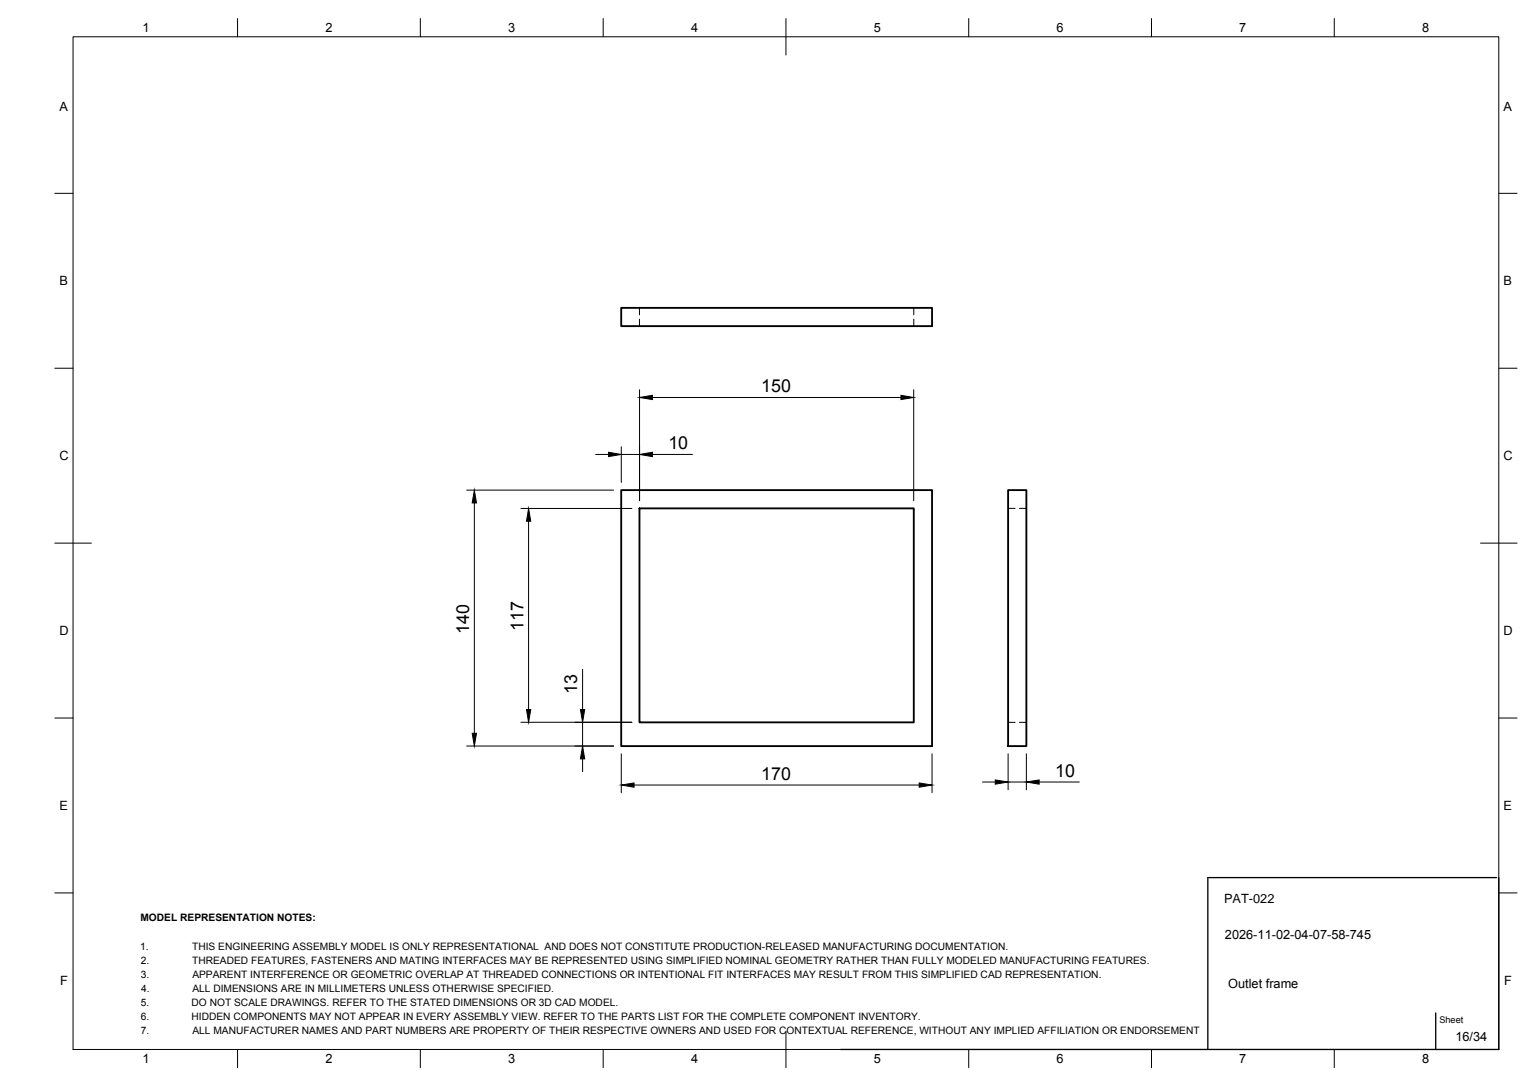
ISO-10303-21;
HEADER;
/* Generated by software containing ST-Developer
 * from STEP Tools, Inc. (www.steptools.com) 
 */

FILE_DESCRIPTION(
/* description */ ('Chute with adjustable gate'),
/* implementation_level */ '2;1');

FILE_NAME(
/* name */ 'Outlet frame.step',
/* time_stamp */ '2026-10-27T10:52:28-07:00',
/* author */ (''),
/* organization */ (''),
/* preprocessor_version */ 'ST-DEVELOPER v20.2',
/* originating_system */ 'Autodesk Translation Framework v15.17.0.0',
/* authorisation */ '');

FILE_SCHEMA (('AUTOMOTIVE_DESIGN { 1 0 10303 214 3 1 1 }'));
ENDSEC;

DATA;
#10=MECHANICAL_DESIGN_GEOMETRIC_PRESENTATION_REPRESENTATION('',(#425),#13094);
#361=SHAPE_REPRESENTATION_RELATIONSHIP('SRR','None',#13262,#393);
#393=ADVANCED_BREP_SHAPE_REPRESENTATION('',(#457),#13071);
#425=STYLED_ITEM('',(#13474),#457);
#457=MANIFOLD_SOLID_BREP('Body1',#7608);
#516=FACE_BOUND('',#1482,.T.);
#517=FACE_BOUND('',#1484,.T.);
#668=PLANE('',#8150);
#669=PLANE('',#8151);
#670=PLANE('',#8152);
#671=PLANE('',#8153);
#672=PLANE('',#8154);
#673=PLANE('',#8155);
#674=PLANE('',#8156);
#675=PLANE('',#8157);
#676=PLANE('',#8158);
#677=PLANE('',#8159);
#1016=FACE_OUTER_BOUND('',#1473,.T.);
#1017=FACE_OUTER_BOUND('',#1474,.T.);
#1018=FACE_OUTER_BOUND('',#1475,.T.);
#1019=FACE_OUTER_BOUND('',#1476,.T.);
#1020=FACE_OUTER_BOUND('',#1477,.T.);
#1021=FACE_OUTER_BOUND('',#1478,.T.);
#1022=FACE_OUTER_BOUND('',#1479,.T.);
#1023=FACE_OUTER_BOUND('',#1480,.T.);
#1024=FACE_OUTER_BOUND('',#1481,.T.);
#1025=FACE_OUTER_BOUND('',#1483,.T.);
#1473=EDGE_LOOP('',(#5618,#5619,#5620,#5621));
#1474=EDGE_LOOP('',(#5622,#5623,#5624,#5625));
#1475=EDGE_LOOP('',(#5626,#5627,#5628,#5629));
#1476=EDGE_LOOP('',(#5630,#5631,#5632,#5633));
#1477=EDGE_LOOP('',(#5634,#5635,#5636,#5637));
#1478=EDGE_LOOP('',(#5638,#5639,#5640,#5641));
#1479=EDGE_LOOP('',(#5642,#5643,#5644,#5645));
#1480=EDGE_LOOP('',(#5646,#5647,#5648,#5649));
#1481=EDGE_LOOP('',(#5650,#5651,#5652,#5653));
#1482=EDGE_LOOP('',(#5654,#5655,#5656,#5657));
#1483=EDGE_LOOP('',(#5658,#5659,#5660,#5661));
#1484=EDGE_LOOP('',(#5662,#5663,#5664,#5665));
#2028=LINE('',#11378,#2805);
#2029=LINE('',#11380,#2806);
#2030=LINE('',#11382,#2807);
#2031=LINE('',#11383,#2808);
#2032=LINE('',#11386,#2809);
#2033=LINE('',#11388,#2810);
#2034=LINE('',#11389,#2811);
#2035=LINE('',#11392,#2812);
#2036=LINE('',#11394,#2813);
#2037=LINE('',#11395,#2814);
#2038=LINE('',#11397,#2815);
#2039=LINE('',#11398,#2816);
#2040=LINE('',#11402,#2817);
#2041=LINE('',#11404,#2818);
#2042=LINE('',#11406,#2819);
#2043=LINE('',#11407,#2820);
#2044=LINE('',#11410,#2821);
#2045=LINE('',#11412,#2822);
#2046=LINE('',#11413,#2823);
#2047=LINE('',#11416,#2824);
#2048=LINE('',#11418,#2825);
#2049=LINE('',#11419,#2826);
#2050=LINE('',#11421,#2827);
#2051=LINE('',#11422,#2828);
#2805=VECTOR('',#9196,1.);
#2806=VECTOR('',#9197,1.);
#2807=VECTOR('',#9198,1.);
#2808=VECTOR('',#9199,1.);
#2809=VECTOR('',#9202,1.);
#2810=VECTOR('',#9203,1.);
#2811=VECTOR('',#9204,1.);
#2812=VECTOR('',#9207,1.);
#2813=VECTOR('',#9208,1.);
#2814=VECTOR('',#9209,1.);
#2815=VECTOR('',#9212,1.);
#2816=VECTOR('',#9213,1.);
#2817=VECTOR('',#9216,1.);
#2818=VECTOR('',#9217,1.);
#2819=VECTOR('',#9218,1.);
#2820=VECTOR('',#9219,1.);
#2821=VECTOR('',#9222,1.);
#2822=VECTOR('',#9223,1.);
#2823=VECTOR('',#9224,1.);
#2824=VECTOR('',#9227,1.);
#2825=VECTOR('',#9228,1.);
#2826=VECTOR('',#9229,1.);
#2827=VECTOR('',#9232,1.);
#2828=VECTOR('',#9233,1.);
#3737=VERTEX_POINT('',#11376);
#3738=VERTEX_POINT('',#11377);
#3739=VERTEX_POINT('',#11379);
#3740=VERTEX_POINT('',#11381);
#3741=VERTEX_POINT('',#11385);
#3742=VERTEX_POINT('',#11387);
#3743=VERTEX_POINT('',#11391);
#3744=VERTEX_POINT('',#11393);
#3745=VERTEX_POINT('',#11400);
#3746=VERTEX_POINT('',#11401);
#3747=VERTEX_POINT('',#11403);
#3748=VERTEX_POINT('',#11405);
#3749=VERTEX_POINT('',#11409);
#3750=VERTEX_POINT('',#11411);
#3751=VERTEX_POINT('',#11415);
#3752=VERTEX_POINT('',#11417);
#4442=EDGE_CURVE('',#3737,#3738,#2028,.T.);
#4443=EDGE_CURVE('',#3739,#3737,#2029,.T.);
#4444=EDGE_CURVE('',#3740,#3739,#2030,.T.);
#4445=EDGE_CURVE('',#3740,#3738,#2031,.T.);
#4446=EDGE_CURVE('',#3738,#3741,#2032,.T.);
#4447=EDGE_CURVE('',#3742,#3740,#2033,.T.);
#4448=EDGE_CURVE('',#3742,#3741,#2034,.T.);
#4449=EDGE_CURVE('',#3741,#3743,#2035,.T.);
#4450=EDGE_CURVE('',#3744,#3742,#2036,.T.);
#4451=EDGE_CURVE('',#3744,#3743,#2037,.T.);
#4452=EDGE_CURVE('',#3743,#3737,#2038,.T.);
#4453=EDGE_CURVE('',#3739,#3744,#2039,.T.);
#4454=EDGE_CURVE('',#3745,#3746,#2040,.T.);
#4455=EDGE_CURVE('',#3746,#3747,#2041,.T.);
#4456=EDGE_CURVE('',#3748,#3747,#2042,.T.);
#4457=EDGE_CURVE('',#3745,#3748,#2043,.T.);
#4458=EDGE_CURVE('',#3749,#3745,#2044,.T.);
#4459=EDGE_CURVE('',#3750,#3748,#2045,.T.);
#4460=EDGE_CURVE('',#3749,#3750,#2046,.T.);
#4461=EDGE_CURVE('',#3751,#3749,#2047,.T.);
#4462=EDGE_CURVE('',#3752,#3750,#2048,.T.);
#4463=EDGE_CURVE('',#3751,#3752,#2049,.T.);
#4464=EDGE_CURVE('',#3746,#3751,#2050,.T.);
#4465=EDGE_CURVE('',#3747,#3752,#2051,.T.);
#5618=ORIENTED_EDGE('',*,*,#4442,.F.);
#5619=ORIENTED_EDGE('',*,*,#4443,.F.);
#5620=ORIENTED_EDGE('',*,*,#4444,.F.);
#5621=ORIENTED_EDGE('',*,*,#4445,.T.);
#5622=ORIENTED_EDGE('',*,*,#4446,.F.);
#5623=ORIENTED_EDGE('',*,*,#4445,.F.);
#5624=ORIENTED_EDGE('',*,*,#4447,.F.);
#5625=ORIENTED_EDGE('',*,*,#4448,.T.);
#5626=ORIENTED_EDGE('',*,*,#4449,.F.);
#5627=ORIENTED_EDGE('',*,*,#4448,.F.);
#5628=ORIENTED_EDGE('',*,*,#4450,.F.);
#5629=ORIENTED_EDGE('',*,*,#4451,.T.);
#5630=ORIENTED_EDGE('',*,*,#4452,.F.);
#5631=ORIENTED_EDGE('',*,*,#4451,.F.);
#5632=ORIENTED_EDGE('',*,*,#4453,.F.);
#5633=ORIENTED_EDGE('',*,*,#4443,.T.);
#5634=ORIENTED_EDGE('',*,*,#4454,.T.);
#5635=ORIENTED_EDGE('',*,*,#4455,.T.);
#5636=ORIENTED_EDGE('',*,*,#4456,.F.);
#5637=ORIENTED_EDGE('',*,*,#4457,.F.);
#5638=ORIENTED_EDGE('',*,*,#4458,.T.);
#5639=ORIENTED_EDGE('',*,*,#4457,.T.);
#5640=ORIENTED_EDGE('',*,*,#4459,.F.);
#5641=ORIENTED_EDGE('',*,*,#4460,.F.);
#5642=ORIENTED_EDGE('',*,*,#4461,.T.);
#5643=ORIENTED_EDGE('',*,*,#4460,.T.);
#5644=ORIENTED_EDGE('',*,*,#4462,.F.);
#5645=ORIENTED_EDGE('',*,*,#4463,.F.);
#5646=ORIENTED_EDGE('',*,*,#4464,.T.);
#5647=ORIENTED_EDGE('',*,*,#4463,.T.);
#5648=ORIENTED_EDGE('',*,*,#4465,.F.);
#5649=ORIENTED_EDGE('',*,*,#4455,.F.);
#5650=ORIENTED_EDGE('',*,*,#4465,.T.);
#5651=ORIENTED_EDGE('',*,*,#4462,.T.);
#5652=ORIENTED_EDGE('',*,*,#4459,.T.);
#5653=ORIENTED_EDGE('',*,*,#4456,.T.);
#5654=ORIENTED_EDGE('',*,*,#4449,.T.);
#5655=ORIENTED_EDGE('',*,*,#4452,.T.);
#5656=ORIENTED_EDGE('',*,*,#4442,.T.);
#5657=ORIENTED_EDGE('',*,*,#4446,.T.);
#5658=ORIENTED_EDGE('',*,*,#4464,.F.);
#5659=ORIENTED_EDGE('',*,*,#4454,.F.);
#5660=ORIENTED_EDGE('',*,*,#4458,.F.);
#5661=ORIENTED_EDGE('',*,*,#4461,.F.);
#5662=ORIENTED_EDGE('',*,*,#4450,.T.);
#5663=ORIENTED_EDGE('',*,*,#4447,.T.);
#5664=ORIENTED_EDGE('',*,*,#4444,.T.);
#5665=ORIENTED_EDGE('',*,*,#4453,.T.);
#7284=ADVANCED_FACE('',(#1016),#668,.F.);
#7285=ADVANCED_FACE('',(#1017),#669,.F.);
#7286=ADVANCED_FACE('',(#1018),#670,.F.);
#7287=ADVANCED_FACE('',(#1019),#671,.F.);
#7288=ADVANCED_FACE('',(#1020),#672,.T.);
#7289=ADVANCED_FACE('',(#1021),#673,.T.);
#7290=ADVANCED_FACE('',(#1022),#674,.T.);
#7291=ADVANCED_FACE('',(#1023),#675,.T.);
#7292=ADVANCED_FACE('',(#1024,#516),#676,.T.);
#7293=ADVANCED_FACE('',(#1025,#517),#677,.F.);
#7608=CLOSED_SHELL('',(#7284,#7285,#7286,#7287,#7288,#7289,#7290,#7291,
#7292,#7293));
#8149=AXIS2_PLACEMENT_3D('',#11374,#9192,#9193);
#8150=AXIS2_PLACEMENT_3D('',#11375,#9194,#9195);
#8151=AXIS2_PLACEMENT_3D('',#11384,#9200,#9201);
#8152=AXIS2_PLACEMENT_3D('',#11390,#9205,#9206);
#8153=AXIS2_PLACEMENT_3D('',#11396,#9210,#9211);
#8154=AXIS2_PLACEMENT_3D('',#11399,#9214,#9215);
#8155=AXIS2_PLACEMENT_3D('',#11408,#9220,#9221);
#8156=AXIS2_PLACEMENT_3D('',#11414,#9225,#9226);
#8157=AXIS2_PLACEMENT_3D('',#11420,#9230,#9231);
#8158=AXIS2_PLACEMENT_3D('',#11423,#9234,#9235);
#8159=AXIS2_PLACEMENT_3D('',#11424,#9236,#9237);
#9192=DIRECTION('axis',(0.,0.,1.));
#9193=DIRECTION('refdir',(1.,0.,0.));
#9194=DIRECTION('center_axis',(0.,0.,-1.));
#9195=DIRECTION('ref_axis',(0.,1.,0.));
#9196=DIRECTION('',(0.,-1.,0.));
#9197=DIRECTION('',(1.,0.,0.));
#9198=DIRECTION('',(0.,1.,0.));
#9199=DIRECTION('',(1.,0.,0.));
#9200=DIRECTION('center_axis',(0.,-1.,0.));
#9201=DIRECTION('ref_axis',(0.,0.,-1.));
#9202=DIRECTION('',(0.,0.,1.));
#9203=DIRECTION('',(0.,0.,-1.));
#9204=DIRECTION('',(1.,0.,0.));
#9205=DIRECTION('center_axis',(0.,0.,1.));
#9206=DIRECTION('ref_axis',(0.,-1.,0.));
#9207=DIRECTION('',(0.,1.,0.));
#9208=DIRECTION('',(0.,-1.,0.));
#9209=DIRECTION('',(1.,0.,0.));
#9210=DIRECTION('center_axis',(0.,1.,0.));
#9211=DIRECTION('ref_axis',(0.,0.,1.));
#9212=DIRECTION('',(0.,0.,-1.));
#9213=DIRECTION('',(0.,0.,1.));
#9214=DIRECTION('center_axis',(0.,0.,1.));
#9215=DIRECTION('ref_axis',(0.,-1.,0.));
#9216=DIRECTION('',(0.,-1.,0.));
#9217=DIRECTION('',(1.,0.,0.));
#9218=DIRECTION('',(0.,-1.,0.));
#9219=DIRECTION('',(1.,0.,0.));
#9220=DIRECTION('center_axis',(0.,1.,0.));
#9221=DIRECTION('ref_axis',(0.,0.,1.));
#9222=DIRECTION('',(0.,0.,1.));
#9223=DIRECTION('',(0.,0.,1.));
#9224=DIRECTION('',(1.,0.,0.));
#9225=DIRECTION('center_axis',(0.,0.,-1.));
#9226=DIRECTION('ref_axis',(0.,1.,0.));
#9227=DIRECTION('',(0.,1.,0.));
#9228=DIRECTION('',(0.,1.,0.));
#9229=DIRECTION('',(1.,0.,0.));
#9230=DIRECTION('center_axis',(0.,-1.,0.));
#9231=DIRECTION('ref_axis',(0.,0.,-1.));
#9232=DIRECTION('',(0.,0.,-1.));
#9233=DIRECTION('',(0.,0.,-1.));
#9234=DIRECTION('center_axis',(1.,0.,0.));
#9235=DIRECTION('ref_axis',(0.,0.,-1.));
#9236=DIRECTION('center_axis',(1.,0.,0.));
#9237=DIRECTION('ref_axis',(0.,0.,-1.));
#11374=CARTESIAN_POINT('',(0.,0.,0.));
#11375=CARTESIAN_POINT('Origin',(-1.1,-7.5,4.3));
#11376=CARTESIAN_POINT('',(0.,7.5,4.3));
#11377=CARTESIAN_POINT('',(0.,-7.5,4.3));
#11378=CARTESIAN_POINT('',(0.,-3.75,4.3));
#11379=CARTESIAN_POINT('',(-1.,7.5,4.3));
#11380=CARTESIAN_POINT('',(-1.1,7.5,4.3));
#11381=CARTESIAN_POINT('',(-1.,-7.5,4.3));
#11382=CARTESIAN_POINT('',(-1.,-3.75,4.3));
#11383=CARTESIAN_POINT('',(-1.1,-7.5,4.3));
#11384=CARTESIAN_POINT('Origin',(-1.1,-7.5,16.));
#11385=CARTESIAN_POINT('',(0.,-7.5,16.));
#11386=CARTESIAN_POINT('',(0.,-7.5,13.));
#11387=CARTESIAN_POINT('',(-1.,-7.5,16.));
#11388=CARTESIAN_POINT('',(-1.,-7.5,13.));
#11389=CARTESIAN_POINT('',(-1.1,-7.5,16.));
#11390=CARTESIAN_POINT('Origin',(-1.1,7.5,16.));
#11391=CARTESIAN_POINT('',(0.,7.5,16.));
#11392=CARTESIAN_POINT('',(0.,3.75,16.));
#11393=CARTESIAN_POINT('',(-1.,7.5,16.));
#11394=CARTESIAN_POINT('',(-1.,3.75,16.));
#11395=CARTESIAN_POINT('',(-1.1,7.5,16.));
#11396=CARTESIAN_POINT('Origin',(-1.1,7.5,4.3));
#11397=CARTESIAN_POINT('',(0.,7.5,7.15));
#11398=CARTESIAN_POINT('',(-1.,7.5,7.15));
#11399=CARTESIAN_POINT('Origin',(-1.,8.5,17.));
#11400=CARTESIAN_POINT('',(-1.,8.5,17.));
#11401=CARTESIAN_POINT('',(-1.,-8.5,17.));
#11402=CARTESIAN_POINT('',(-1.,8.5,17.));
#11403=CARTESIAN_POINT('',(0.,-8.5,17.));
#11404=CARTESIAN_POINT('',(-1.,-8.5,17.));
#11405=CARTESIAN_POINT('',(0.,8.5,17.));
#11406=CARTESIAN_POINT('',(0.,8.5,17.));
#11407=CARTESIAN_POINT('',(-1.,8.5,17.));
#11408=CARTESIAN_POINT('Origin',(-1.,8.5,3.));
#11409=CARTESIAN_POINT('',(-1.,8.5,3.));
#11410=CARTESIAN_POINT('',(-1.,8.5,3.));
#11411=CARTESIAN_POINT('',(0.,8.5,3.));
#11412=CARTESIAN_POINT('',(0.,8.5,3.));
#11413=CARTESIAN_POINT('',(-1.,8.5,3.));
#11414=CARTESIAN_POINT('Origin',(-1.,-8.5,3.));
#11415=CARTESIAN_POINT('',(-1.,-8.5,3.));
#11416=CARTESIAN_POINT('',(-1.,-8.5,3.));
#11417=CARTESIAN_POINT('',(0.,-8.5,3.));
#11418=CARTESIAN_POINT('',(0.,-8.5,3.));
#11419=CARTESIAN_POINT('',(-1.,-8.5,3.));
#11420=CARTESIAN_POINT('Origin',(-1.,-8.5,17.));
#11421=CARTESIAN_POINT('',(-1.,-8.5,17.));
#11422=CARTESIAN_POINT('',(0.,-8.5,17.));
#11423=CARTESIAN_POINT('Origin',(0.,0.,10.));
#11424=CARTESIAN_POINT('Origin',(-1.,0.,10.));
#13034=UNCERTAINTY_MEASURE_WITH_UNIT(LENGTH_MEASURE(0.001),#13095,
'DISTANCE_ACCURACY_VALUE',
'Maximum model space distance between geometric entities at asserted c
onnectivities');
#13057=UNCERTAINTY_MEASURE_WITH_UNIT(LENGTH_MEASURE(0.001),#13095,
'DISTANCE_ACCURACY_VALUE',
'Maximum model space distance between geometric entities at asserted c
onnectivities');
#13071=(
GEOMETRIC_REPRESENTATION_CONTEXT(3)
GLOBAL_UNCERTAINTY_ASSIGNED_CONTEXT((#13034))
GLOBAL_UNIT_ASSIGNED_CONTEXT((#13095,#13097,#13098))
REPRESENTATION_CONTEXT('','3D')
);
#13094=(
GEOMETRIC_REPRESENTATION_CONTEXT(3)
GLOBAL_UNCERTAINTY_ASSIGNED_CONTEXT((#13057))
GLOBAL_UNIT_ASSIGNED_CONTEXT((#13095,#13097,#13098))
REPRESENTATION_CONTEXT('','3D')
);
#13095=(
LENGTH_UNIT()
NAMED_UNIT(*)
SI_UNIT(.CENTI.,.METRE.)
);
#13097=(
NAMED_UNIT(*)
PLANE_ANGLE_UNIT()
SI_UNIT($,.RADIAN.)
);
#13098=(
NAMED_UNIT(*)
SI_UNIT($,.STERADIAN.)
SOLID_ANGLE_UNIT()
);
#13112=SHAPE_DEFINITION_REPRESENTATION(#13148,#13262);
#13148=PRODUCT_DEFINITION_SHAPE('',$,#13299);
#13262=SHAPE_REPRESENTATION('',(#8149),#13071);
#13285=PRODUCT_DEFINITION_CONTEXT('part definition',#13395,'design');
#13299=PRODUCT_DEFINITION('Outlet frame','Outlet frame',#13335,#13285);
#13335=PRODUCT_DEFINITION_FORMATION('',$,#13410);
#13395=APPLICATION_CONTEXT(
'Core Data for Automotive Mechanical Design Process');
#13396=PRODUCT_CONTEXT('part definition',#13395,'mechanical');
#13410=PRODUCT('Outlet frame','Outlet frame','Outlet frame',(#13396));
#13468=COLOUR_RGB('Dark Blue',0.08,0.2,0.34);
#13469=FILL_AREA_STYLE_COLOUR('',#13468);
#13470=FILL_AREA_STYLE('',(#13469));
#13471=SURFACE_STYLE_FILL_AREA(#13470);
#13472=SURFACE_SIDE_STYLE('',(#13471));
#13473=SURFACE_STYLE_USAGE(.BOTH.,#13472);
#13474=PRESENTATION_STYLE_ASSIGNMENT((#13473));
ENDSEC;
END-ISO-10303-21;
